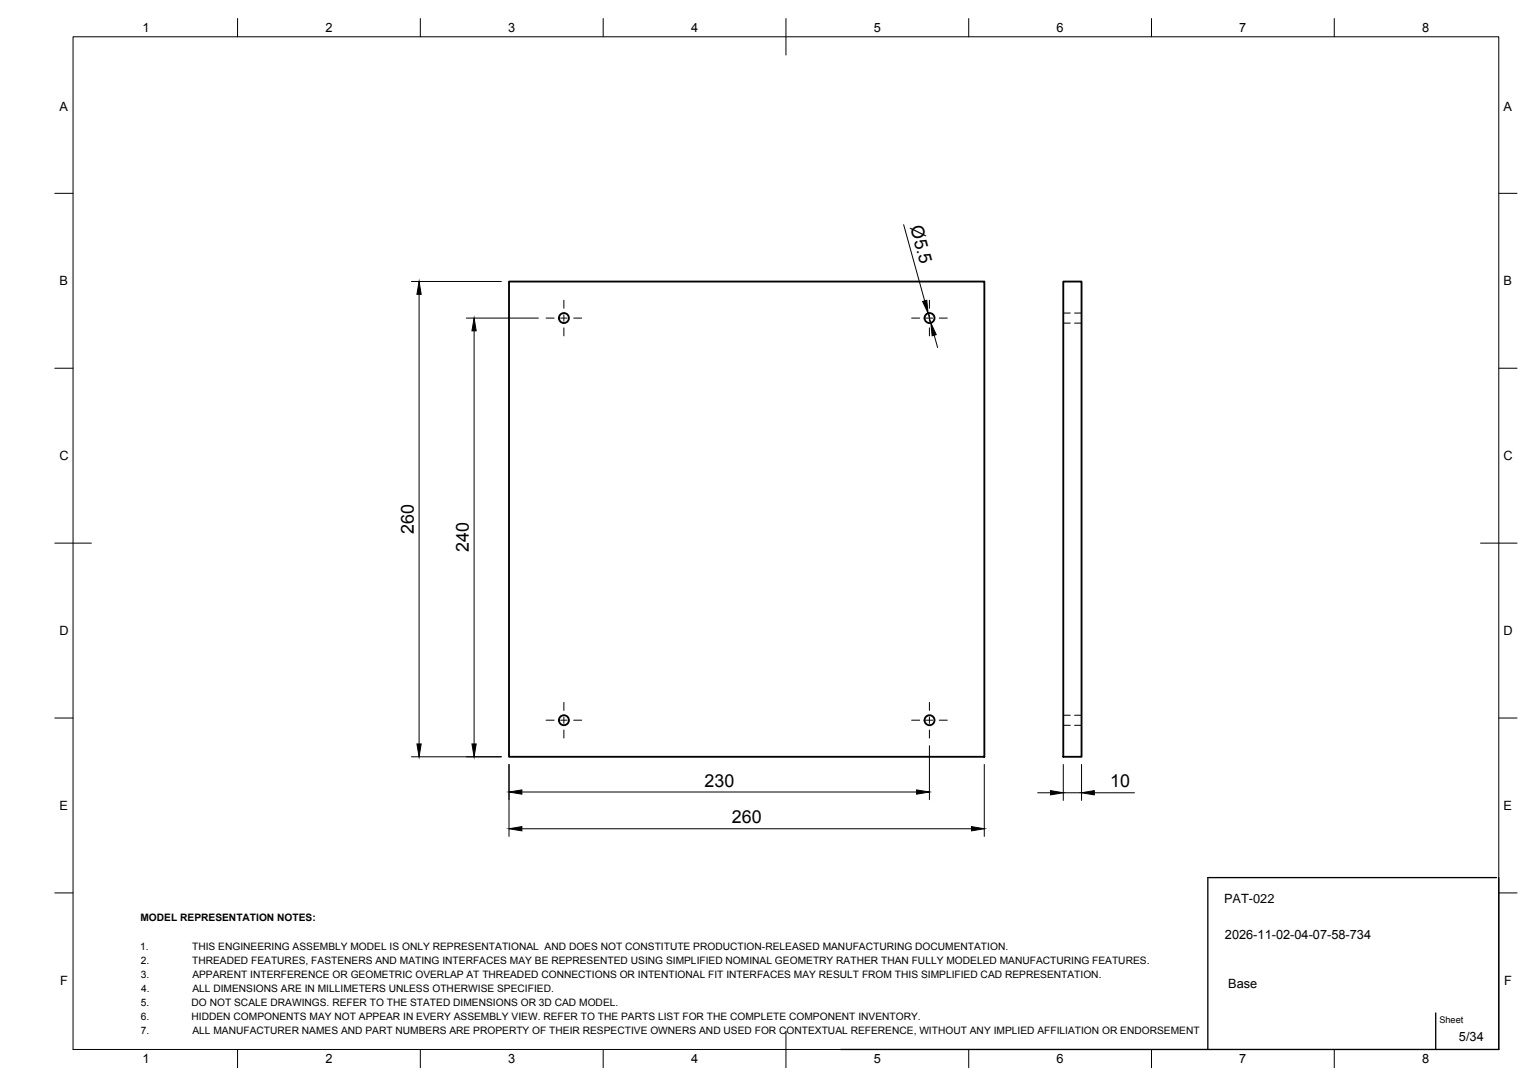
ISO-10303-21;
HEADER;
/* Generated by software containing ST-Developer
 * from STEP Tools, Inc. (www.steptools.com) 
 */

FILE_DESCRIPTION(
/* description */ ('Chute with adjustable gate'),
/* implementation_level */ '2;1');

FILE_NAME(
/* name */ 'Base.step',
/* time_stamp */ '2026-10-27T10:52:28-07:00',
/* author */ (''),
/* organization */ (''),
/* preprocessor_version */ 'ST-DEVELOPER v20.2',
/* originating_system */ 'Autodesk Translation Framework v15.17.0.0',
/* authorisation */ '');

FILE_SCHEMA (('AUTOMOTIVE_DESIGN { 1 0 10303 214 3 1 1 }'));
ENDSEC;

DATA;
#10=MECHANICAL_DESIGN_GEOMETRIC_PRESENTATION_REPRESENTATION('',(#414),#13094);
#350=SHAPE_REPRESENTATION_RELATIONSHIP('SRR','None',#13251,#382);
#382=ADVANCED_BREP_SHAPE_REPRESENTATION('',(#446),#13060);
#414=STYLED_ITEM('',(#13474),#446);
#446=MANIFOLD_SOLID_BREP('Body1',#7597);
#474=FACE_BOUND('',#1338,.T.);
#475=FACE_BOUND('',#1339,.T.);
#476=FACE_BOUND('',#1340,.T.);
#477=FACE_BOUND('',#1341,.T.);
#478=FACE_BOUND('',#1343,.T.);
#479=FACE_BOUND('',#1344,.T.);
#480=FACE_BOUND('',#1345,.T.);
#481=FACE_BOUND('',#1346,.T.);
#590=PLANE('',#8001);
#591=PLANE('',#8002);
#592=PLANE('',#8003);
#593=PLANE('',#8004);
#594=PLANE('',#8005);
#595=PLANE('',#8006);
#914=FACE_OUTER_BOUND('',#1329,.T.);
#915=FACE_OUTER_BOUND('',#1330,.T.);
#916=FACE_OUTER_BOUND('',#1331,.T.);
#917=FACE_OUTER_BOUND('',#1332,.T.);
#918=FACE_OUTER_BOUND('',#1333,.T.);
#919=FACE_OUTER_BOUND('',#1334,.T.);
#920=FACE_OUTER_BOUND('',#1335,.T.);
#921=FACE_OUTER_BOUND('',#1336,.T.);
#922=FACE_OUTER_BOUND('',#1337,.T.);
#923=FACE_OUTER_BOUND('',#1342,.T.);
#1329=EDGE_LOOP('',(#5186,#5187,#5188,#5189));
#1330=EDGE_LOOP('',(#5190,#5191,#5192,#5193));
#1331=EDGE_LOOP('',(#5194,#5195,#5196,#5197));
#1332=EDGE_LOOP('',(#5198,#5199,#5200,#5201));
#1333=EDGE_LOOP('',(#5202,#5203,#5204,#5205));
#1334=EDGE_LOOP('',(#5206,#5207,#5208,#5209));
#1335=EDGE_LOOP('',(#5210,#5211,#5212,#5213));
#1336=EDGE_LOOP('',(#5214,#5215,#5216,#5217));
#1337=EDGE_LOOP('',(#5218,#5219,#5220,#5221));
#1338=EDGE_LOOP('',(#5222));
#1339=EDGE_LOOP('',(#5223));
#1340=EDGE_LOOP('',(#5224));
#1341=EDGE_LOOP('',(#5225));
#1342=EDGE_LOOP('',(#5226,#5227,#5228,#5229));
#1343=EDGE_LOOP('',(#5230));
#1344=EDGE_LOOP('',(#5231));
#1345=EDGE_LOOP('',(#5232));
#1346=EDGE_LOOP('',(#5233));
#1860=LINE('',#10906,#2637);
#1861=LINE('',#10912,#2638);
#1862=LINE('',#10918,#2639);
#1863=LINE('',#10924,#2640);
#1864=LINE('',#10929,#2641);
#1865=LINE('',#10931,#2642);
#1866=LINE('',#10933,#2643);
#1867=LINE('',#10934,#2644);
#1868=LINE('',#10937,#2645);
#1869=LINE('',#10939,#2646);
#1870=LINE('',#10940,#2647);
#1871=LINE('',#10943,#2648);
#1872=LINE('',#10945,#2649);
#1873=LINE('',#10946,#2650);
#1874=LINE('',#10948,#2651);
#1875=LINE('',#10949,#2652);
#2637=VECTOR('',#8708,0.274999999999999);
#2638=VECTOR('',#8715,0.275);
#2639=VECTOR('',#8722,0.275);
#2640=VECTOR('',#8729,0.274999999999999);
#2641=VECTOR('',#8734,1.);
#2642=VECTOR('',#8735,1.);
#2643=VECTOR('',#8736,1.);
#2644=VECTOR('',#8737,1.);
#2645=VECTOR('',#8740,1.);
#2646=VECTOR('',#8741,1.);
#2647=VECTOR('',#8742,1.);
#2648=VECTOR('',#8745,1.);
#2649=VECTOR('',#8746,1.);
#2650=VECTOR('',#8747,1.);
#2651=VECTOR('',#8750,1.);
#2652=VECTOR('',#8751,1.);
#3414=CIRCLE('',#7990,0.274999999999999);
#3415=CIRCLE('',#7991,0.274999999999999);
#3416=CIRCLE('',#7993,0.275);
#3417=CIRCLE('',#7994,0.275);
#3418=CIRCLE('',#7996,0.275);
#3419=CIRCLE('',#7997,0.275);
#3420=CIRCLE('',#7999,0.274999999999999);
#3421=CIRCLE('',#8000,0.274999999999999);
#3593=VERTEX_POINT('',#10903);
#3594=VERTEX_POINT('',#10905);
#3595=VERTEX_POINT('',#10909);
#3596=VERTEX_POINT('',#10911);
#3597=VERTEX_POINT('',#10915);
#3598=VERTEX_POINT('',#10917);
#3599=VERTEX_POINT('',#10921);
#3600=VERTEX_POINT('',#10923);
#3601=VERTEX_POINT('',#10927);
#3602=VERTEX_POINT('',#10928);
#3603=VERTEX_POINT('',#10930);
#3604=VERTEX_POINT('',#10932);
#3605=VERTEX_POINT('',#10936);
#3606=VERTEX_POINT('',#10938);
#3607=VERTEX_POINT('',#10942);
#3608=VERTEX_POINT('',#10944);
#4226=EDGE_CURVE('',#3593,#3593,#3414,.T.);
#4227=EDGE_CURVE('',#3593,#3594,#1860,.T.);
#4228=EDGE_CURVE('',#3594,#3594,#3415,.T.);
#4229=EDGE_CURVE('',#3595,#3595,#3416,.T.);
#4230=EDGE_CURVE('',#3595,#3596,#1861,.T.);
#4231=EDGE_CURVE('',#3596,#3596,#3417,.T.);
#4232=EDGE_CURVE('',#3597,#3597,#3418,.T.);
#4233=EDGE_CURVE('',#3597,#3598,#1862,.T.);
#4234=EDGE_CURVE('',#3598,#3598,#3419,.T.);
#4235=EDGE_CURVE('',#3599,#3599,#3420,.T.);
#4236=EDGE_CURVE('',#3599,#3600,#1863,.T.);
#4237=EDGE_CURVE('',#3600,#3600,#3421,.T.);
#4238=EDGE_CURVE('',#3601,#3602,#1864,.T.);
#4239=EDGE_CURVE('',#3602,#3603,#1865,.T.);
#4240=EDGE_CURVE('',#3604,#3603,#1866,.T.);
#4241=EDGE_CURVE('',#3601,#3604,#1867,.T.);
#4242=EDGE_CURVE('',#3605,#3601,#1868,.T.);
#4243=EDGE_CURVE('',#3606,#3604,#1869,.T.);
#4244=EDGE_CURVE('',#3605,#3606,#1870,.T.);
#4245=EDGE_CURVE('',#3607,#3605,#1871,.T.);
#4246=EDGE_CURVE('',#3608,#3606,#1872,.T.);
#4247=EDGE_CURVE('',#3607,#3608,#1873,.T.);
#4248=EDGE_CURVE('',#3602,#3607,#1874,.T.);
#4249=EDGE_CURVE('',#3603,#3608,#1875,.T.);
#5186=ORIENTED_EDGE('',*,*,#4226,.F.);
#5187=ORIENTED_EDGE('',*,*,#4227,.T.);
#5188=ORIENTED_EDGE('',*,*,#4228,.F.);
#5189=ORIENTED_EDGE('',*,*,#4227,.F.);
#5190=ORIENTED_EDGE('',*,*,#4229,.F.);
#5191=ORIENTED_EDGE('',*,*,#4230,.T.);
#5192=ORIENTED_EDGE('',*,*,#4231,.F.);
#5193=ORIENTED_EDGE('',*,*,#4230,.F.);
#5194=ORIENTED_EDGE('',*,*,#4232,.F.);
#5195=ORIENTED_EDGE('',*,*,#4233,.T.);
#5196=ORIENTED_EDGE('',*,*,#4234,.F.);
#5197=ORIENTED_EDGE('',*,*,#4233,.F.);
#5198=ORIENTED_EDGE('',*,*,#4235,.F.);
#5199=ORIENTED_EDGE('',*,*,#4236,.T.);
#5200=ORIENTED_EDGE('',*,*,#4237,.F.);
#5201=ORIENTED_EDGE('',*,*,#4236,.F.);
#5202=ORIENTED_EDGE('',*,*,#4238,.T.);
#5203=ORIENTED_EDGE('',*,*,#4239,.T.);
#5204=ORIENTED_EDGE('',*,*,#4240,.F.);
#5205=ORIENTED_EDGE('',*,*,#4241,.F.);
#5206=ORIENTED_EDGE('',*,*,#4242,.T.);
#5207=ORIENTED_EDGE('',*,*,#4241,.T.);
#5208=ORIENTED_EDGE('',*,*,#4243,.F.);
#5209=ORIENTED_EDGE('',*,*,#4244,.F.);
#5210=ORIENTED_EDGE('',*,*,#4245,.T.);
#5211=ORIENTED_EDGE('',*,*,#4244,.T.);
#5212=ORIENTED_EDGE('',*,*,#4246,.F.);
#5213=ORIENTED_EDGE('',*,*,#4247,.F.);
#5214=ORIENTED_EDGE('',*,*,#4248,.T.);
#5215=ORIENTED_EDGE('',*,*,#4247,.T.);
#5216=ORIENTED_EDGE('',*,*,#4249,.F.);
#5217=ORIENTED_EDGE('',*,*,#4239,.F.);
#5218=ORIENTED_EDGE('',*,*,#4249,.T.);
#5219=ORIENTED_EDGE('',*,*,#4246,.T.);
#5220=ORIENTED_EDGE('',*,*,#4243,.T.);
#5221=ORIENTED_EDGE('',*,*,#4240,.T.);
#5222=ORIENTED_EDGE('',*,*,#4228,.T.);
#5223=ORIENTED_EDGE('',*,*,#4231,.T.);
#5224=ORIENTED_EDGE('',*,*,#4234,.T.);
#5225=ORIENTED_EDGE('',*,*,#4237,.T.);
#5226=ORIENTED_EDGE('',*,*,#4248,.F.);
#5227=ORIENTED_EDGE('',*,*,#4238,.F.);
#5228=ORIENTED_EDGE('',*,*,#4242,.F.);
#5229=ORIENTED_EDGE('',*,*,#4245,.F.);
#5230=ORIENTED_EDGE('',*,*,#4226,.T.);
#5231=ORIENTED_EDGE('',*,*,#4229,.T.);
#5232=ORIENTED_EDGE('',*,*,#4232,.T.);
#5233=ORIENTED_EDGE('',*,*,#4235,.T.);
#7106=CYLINDRICAL_SURFACE('',#7989,0.274999999999999);
#7107=CYLINDRICAL_SURFACE('',#7992,0.275);
#7108=CYLINDRICAL_SURFACE('',#7995,0.275);
#7109=CYLINDRICAL_SURFACE('',#7998,0.274999999999999);
#7182=ADVANCED_FACE('',(#914),#7106,.F.);
#7183=ADVANCED_FACE('',(#915),#7107,.F.);
#7184=ADVANCED_FACE('',(#916),#7108,.F.);
#7185=ADVANCED_FACE('',(#917),#7109,.F.);
#7186=ADVANCED_FACE('',(#918),#590,.T.);
#7187=ADVANCED_FACE('',(#919),#591,.T.);
#7188=ADVANCED_FACE('',(#920),#592,.T.);
#7189=ADVANCED_FACE('',(#921),#593,.T.);
#7190=ADVANCED_FACE('',(#922,#474,#475,#476,#477),#594,.T.);
#7191=ADVANCED_FACE('',(#923,#478,#479,#480,#481),#595,.F.);
#7597=CLOSED_SHELL('',(#7182,#7183,#7184,#7185,#7186,#7187,#7188,#7189,
#7190,#7191));
#7988=AXIS2_PLACEMENT_3D('',#10901,#8702,#8703);
#7989=AXIS2_PLACEMENT_3D('',#10902,#8704,#8705);
#7990=AXIS2_PLACEMENT_3D('',#10904,#8706,#8707);
#7991=AXIS2_PLACEMENT_3D('',#10907,#8709,#8710);
#7992=AXIS2_PLACEMENT_3D('',#10908,#8711,#8712);
#7993=AXIS2_PLACEMENT_3D('',#10910,#8713,#8714);
#7994=AXIS2_PLACEMENT_3D('',#10913,#8716,#8717);
#7995=AXIS2_PLACEMENT_3D('',#10914,#8718,#8719);
#7996=AXIS2_PLACEMENT_3D('',#10916,#8720,#8721);
#7997=AXIS2_PLACEMENT_3D('',#10919,#8723,#8724);
#7998=AXIS2_PLACEMENT_3D('',#10920,#8725,#8726);
#7999=AXIS2_PLACEMENT_3D('',#10922,#8727,#8728);
#8000=AXIS2_PLACEMENT_3D('',#10925,#8730,#8731);
#8001=AXIS2_PLACEMENT_3D('',#10926,#8732,#8733);
#8002=AXIS2_PLACEMENT_3D('',#10935,#8738,#8739);
#8003=AXIS2_PLACEMENT_3D('',#10941,#8743,#8744);
#8004=AXIS2_PLACEMENT_3D('',#10947,#8748,#8749);
#8005=AXIS2_PLACEMENT_3D('',#10950,#8752,#8753);
#8006=AXIS2_PLACEMENT_3D('',#10951,#8754,#8755);
#8702=DIRECTION('axis',(0.,0.,1.));
#8703=DIRECTION('refdir',(1.,0.,0.));
#8704=DIRECTION('center_axis',(0.,0.,1.));
#8705=DIRECTION('ref_axis',(1.,0.,0.));
#8706=DIRECTION('center_axis',(0.,0.,1.));
#8707=DIRECTION('ref_axis',(1.,0.,0.));
#8708=DIRECTION('',(0.,0.,1.));
#8709=DIRECTION('center_axis',(0.,0.,-1.));
#8710=DIRECTION('ref_axis',(1.,0.,0.));
#8711=DIRECTION('center_axis',(0.,0.,1.));
#8712=DIRECTION('ref_axis',(1.,0.,0.));
#8713=DIRECTION('center_axis',(0.,0.,1.));
#8714=DIRECTION('ref_axis',(1.,0.,0.));
#8715=DIRECTION('',(0.,0.,1.));
#8716=DIRECTION('center_axis',(0.,0.,-1.));
#8717=DIRECTION('ref_axis',(1.,0.,0.));
#8718=DIRECTION('center_axis',(0.,0.,1.));
#8719=DIRECTION('ref_axis',(1.,0.,0.));
#8720=DIRECTION('center_axis',(0.,0.,1.));
#8721=DIRECTION('ref_axis',(1.,0.,0.));
#8722=DIRECTION('',(0.,0.,1.));
#8723=DIRECTION('center_axis',(0.,0.,-1.));
#8724=DIRECTION('ref_axis',(1.,0.,0.));
#8725=DIRECTION('center_axis',(0.,0.,1.));
#8726=DIRECTION('ref_axis',(1.,0.,0.));
#8727=DIRECTION('center_axis',(0.,0.,1.));
#8728=DIRECTION('ref_axis',(1.,0.,0.));
#8729=DIRECTION('',(0.,0.,1.));
#8730=DIRECTION('center_axis',(0.,0.,-1.));
#8731=DIRECTION('ref_axis',(1.,0.,0.));
#8732=DIRECTION('center_axis',(0.,1.,0.));
#8733=DIRECTION('ref_axis',(-1.,0.,0.));
#8734=DIRECTION('',(-1.,0.,0.));
#8735=DIRECTION('',(0.,0.,1.));
#8736=DIRECTION('',(-1.,0.,0.));
#8737=DIRECTION('',(0.,0.,1.));
#8738=DIRECTION('center_axis',(1.,0.,0.));
#8739=DIRECTION('ref_axis',(0.,1.,0.));
#8740=DIRECTION('',(0.,1.,0.));
#8741=DIRECTION('',(0.,1.,0.));
#8742=DIRECTION('',(0.,0.,1.));
#8743=DIRECTION('center_axis',(0.,-1.,0.));
#8744=DIRECTION('ref_axis',(1.,0.,0.));
#8745=DIRECTION('',(1.,0.,0.));
#8746=DIRECTION('',(1.,0.,0.));
#8747=DIRECTION('',(0.,0.,1.));
#8748=DIRECTION('center_axis',(-1.,0.,0.));
#8749=DIRECTION('ref_axis',(0.,-1.,0.));
#8750=DIRECTION('',(0.,-1.,0.));
#8751=DIRECTION('',(0.,-1.,0.));
#8752=DIRECTION('center_axis',(0.,0.,1.));
#8753=DIRECTION('ref_axis',(1.,0.,0.));
#8754=DIRECTION('center_axis',(0.,0.,1.));
#8755=DIRECTION('ref_axis',(1.,0.,0.));
#10901=CARTESIAN_POINT('',(0.,0.,0.));
#10902=CARTESIAN_POINT('Origin',(23.,-11.,-1.1));
#10903=CARTESIAN_POINT('',(22.725,-11.,-1.));
#10904=CARTESIAN_POINT('Origin',(23.,-11.,-1.));
#10905=CARTESIAN_POINT('',(22.725,-11.,0.));
#10906=CARTESIAN_POINT('',(22.725,-11.,-1.1));
#10907=CARTESIAN_POINT('Origin',(23.,-11.,0.));
#10908=CARTESIAN_POINT('Origin',(3.,11.,-1.1));
#10909=CARTESIAN_POINT('',(2.725,11.,-1.));
#10910=CARTESIAN_POINT('Origin',(3.,11.,-1.));
#10911=CARTESIAN_POINT('',(2.725,11.,0.));
#10912=CARTESIAN_POINT('',(2.725,11.,-1.1));
#10913=CARTESIAN_POINT('Origin',(3.,11.,0.));
#10914=CARTESIAN_POINT('Origin',(3.,-11.,-1.1));
#10915=CARTESIAN_POINT('',(2.725,-11.,-1.));
#10916=CARTESIAN_POINT('Origin',(3.,-11.,-1.));
#10917=CARTESIAN_POINT('',(2.725,-11.,0.));
#10918=CARTESIAN_POINT('',(2.725,-11.,-1.1));
#10919=CARTESIAN_POINT('Origin',(3.,-11.,0.));
#10920=CARTESIAN_POINT('Origin',(23.,11.,-1.1));
#10921=CARTESIAN_POINT('',(22.725,11.,-1.));
#10922=CARTESIAN_POINT('Origin',(23.,11.,-1.));
#10923=CARTESIAN_POINT('',(22.725,11.,0.));
#10924=CARTESIAN_POINT('',(22.725,11.,-1.1));
#10925=CARTESIAN_POINT('Origin',(23.,11.,0.));
#10926=CARTESIAN_POINT('Origin',(26.,13.,-1.));
#10927=CARTESIAN_POINT('',(26.,13.,-1.));
#10928=CARTESIAN_POINT('',(0.,13.,-1.));
#10929=CARTESIAN_POINT('',(26.,13.,-1.));
#10930=CARTESIAN_POINT('',(0.,13.,0.));
#10931=CARTESIAN_POINT('',(0.,13.,-1.));
#10932=CARTESIAN_POINT('',(26.,13.,0.));
#10933=CARTESIAN_POINT('',(26.,13.,0.));
#10934=CARTESIAN_POINT('',(26.,13.,-1.));
#10935=CARTESIAN_POINT('Origin',(26.,-13.,-1.));
#10936=CARTESIAN_POINT('',(26.,-13.,-1.));
#10937=CARTESIAN_POINT('',(26.,-13.,-1.));
#10938=CARTESIAN_POINT('',(26.,-13.,0.));
#10939=CARTESIAN_POINT('',(26.,-13.,0.));
#10940=CARTESIAN_POINT('',(26.,-13.,-1.));
#10941=CARTESIAN_POINT('Origin',(0.,-13.,-1.));
#10942=CARTESIAN_POINT('',(0.,-13.,-1.));
#10943=CARTESIAN_POINT('',(0.,-13.,-1.));
#10944=CARTESIAN_POINT('',(0.,-13.,0.));
#10945=CARTESIAN_POINT('',(0.,-13.,0.));
#10946=CARTESIAN_POINT('',(0.,-13.,-1.));
#10947=CARTESIAN_POINT('Origin',(0.,13.,-1.));
#10948=CARTESIAN_POINT('',(0.,13.,-1.));
#10949=CARTESIAN_POINT('',(0.,13.,0.));
#10950=CARTESIAN_POINT('Origin',(13.,0.,0.));
#10951=CARTESIAN_POINT('Origin',(13.,0.,-1.));
#13023=UNCERTAINTY_MEASURE_WITH_UNIT(LENGTH_MEASURE(0.001),#13095,
'DISTANCE_ACCURACY_VALUE',
'Maximum model space distance between geometric entities at asserted c
onnectivities');
#13057=UNCERTAINTY_MEASURE_WITH_UNIT(LENGTH_MEASURE(0.001),#13095,
'DISTANCE_ACCURACY_VALUE',
'Maximum model space distance between geometric entities at asserted c
onnectivities');
#13060=(
GEOMETRIC_REPRESENTATION_CONTEXT(3)
GLOBAL_UNCERTAINTY_ASSIGNED_CONTEXT((#13023))
GLOBAL_UNIT_ASSIGNED_CONTEXT((#13095,#13097,#13098))
REPRESENTATION_CONTEXT('','3D')
);
#13094=(
GEOMETRIC_REPRESENTATION_CONTEXT(3)
GLOBAL_UNCERTAINTY_ASSIGNED_CONTEXT((#13057))
GLOBAL_UNIT_ASSIGNED_CONTEXT((#13095,#13097,#13098))
REPRESENTATION_CONTEXT('','3D')
);
#13095=(
LENGTH_UNIT()
NAMED_UNIT(*)
SI_UNIT(.CENTI.,.METRE.)
);
#13097=(
NAMED_UNIT(*)
PLANE_ANGLE_UNIT()
SI_UNIT($,.RADIAN.)
);
#13098=(
NAMED_UNIT(*)
SI_UNIT($,.STERADIAN.)
SOLID_ANGLE_UNIT()
);
#13101=SHAPE_DEFINITION_REPRESENTATION(#13137,#13251);
#13137=PRODUCT_DEFINITION_SHAPE('',$,#13288);
#13251=SHAPE_REPRESENTATION('',(#7988),#13060);
#13285=PRODUCT_DEFINITION_CONTEXT('part definition',#13395,'design');
#13288=PRODUCT_DEFINITION('Base','Base',#13324,#13285);
#13324=PRODUCT_DEFINITION_FORMATION('',$,#13399);
#13395=APPLICATION_CONTEXT(
'Core Data for Automotive Mechanical Design Process');
#13396=PRODUCT_CONTEXT('part definition',#13395,'mechanical');
#13399=PRODUCT('Base','Base','Base',(#13396));
#13468=COLOUR_RGB('Dark Blue',0.08,0.2,0.34);
#13469=FILL_AREA_STYLE_COLOUR('',#13468);
#13470=FILL_AREA_STYLE('',(#13469));
#13471=SURFACE_STYLE_FILL_AREA(#13470);
#13472=SURFACE_SIDE_STYLE('',(#13471));
#13473=SURFACE_STYLE_USAGE(.BOTH.,#13472);
#13474=PRESENTATION_STYLE_ASSIGNMENT((#13473));
ENDSEC;
END-ISO-10303-21;
